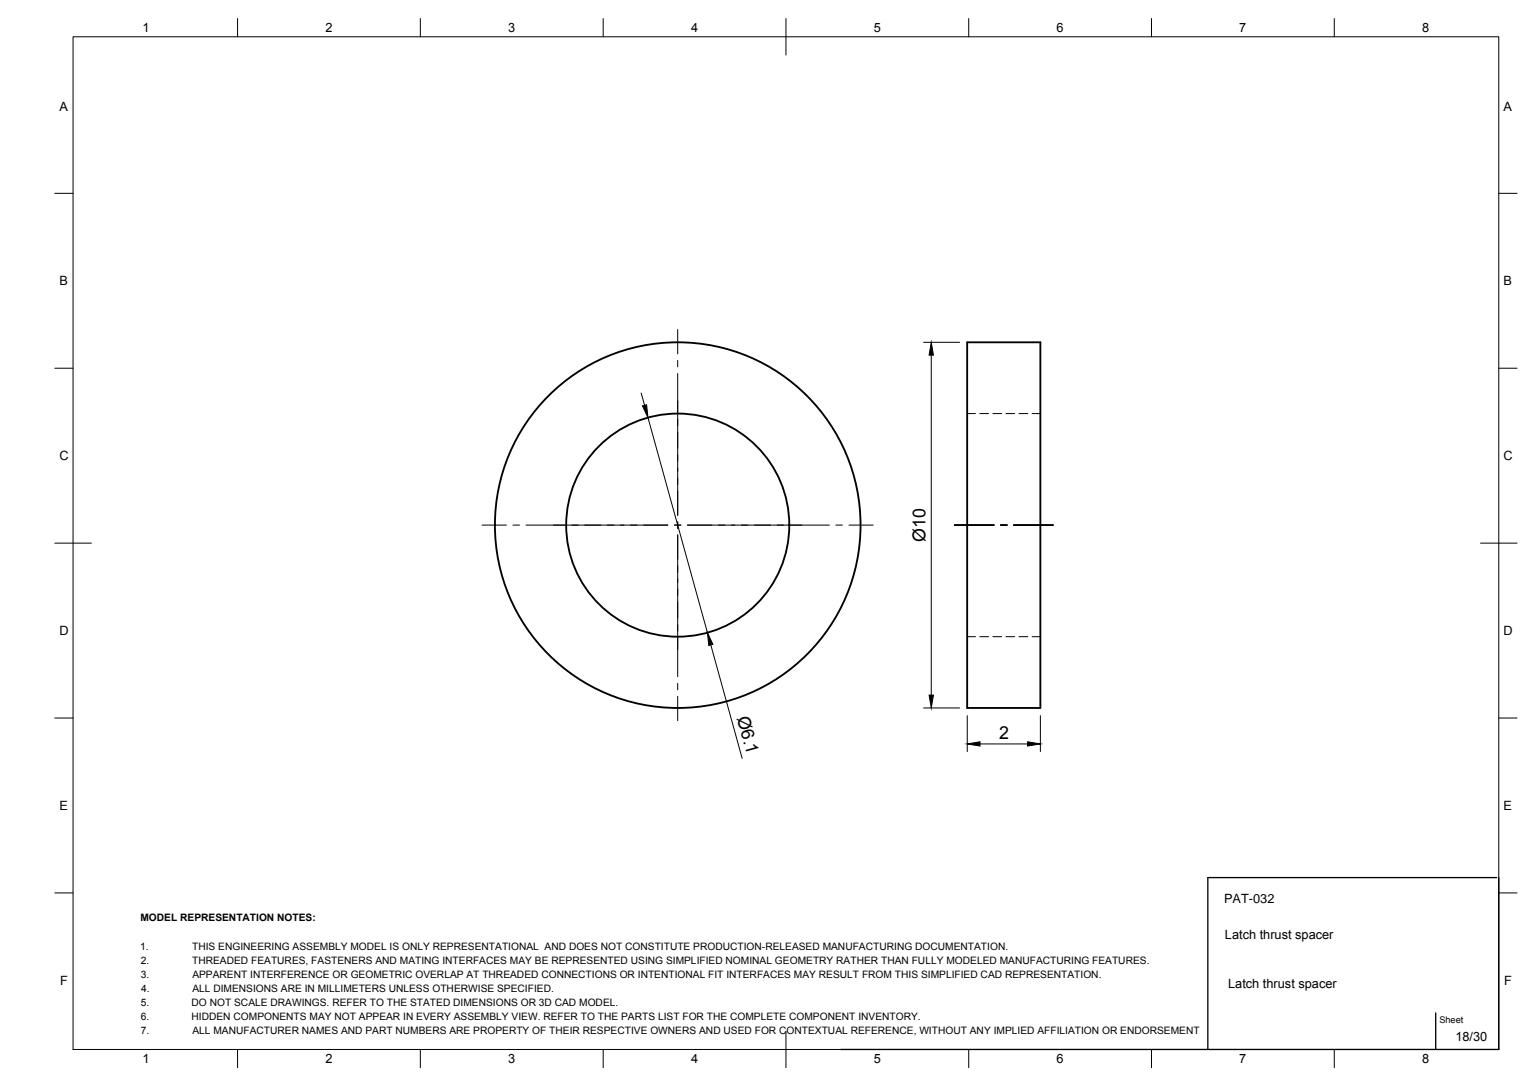
ISO-10303-21;
HEADER;
/* Generated by software containing ST-Developer
 * from STEP Tools, Inc. (www.steptools.com) 
 */

FILE_DESCRIPTION(
/* description */ ('Drill jig with bushing plate'),
/* implementation_level */ '2;1');

FILE_NAME(
/* name */ 'Latch thrust spacer.step',
/* time_stamp */ '2026-10-27T10:51:08-07:00',
/* author */ (''),
/* organization */ (''),
/* preprocessor_version */ 'ST-DEVELOPER v20.2',
/* originating_system */ 'Autodesk Translation Framework v15.17.0.0',
/* authorisation */ '');

FILE_SCHEMA (('AUTOMOTIVE_DESIGN { 1 0 10303 214 3 1 1 }'));
ENDSEC;

DATA;
#10=MECHANICAL_DESIGN_GEOMETRIC_PRESENTATION_REPRESENTATION('',(#236),#6638);
#188=SHAPE_REPRESENTATION_RELATIONSHIP('SRR','None',#6752,#212);
#212=ADVANCED_BREP_SHAPE_REPRESENTATION('',(#260),#6625);
#236=STYLED_ITEM('',(#6936),#260);
#260=MANIFOLD_SOLID_BREP('Body1',#3603);
#339=FACE_BOUND('',#903,.T.);
#340=FACE_BOUND('',#905,.T.);
#438=PLANE('',#4120);
#439=PLANE('',#4121);
#616=FACE_OUTER_BOUND('',#900,.T.);
#617=FACE_OUTER_BOUND('',#901,.T.);
#618=FACE_OUTER_BOUND('',#902,.T.);
#619=FACE_OUTER_BOUND('',#904,.T.);
#900=EDGE_LOOP('',(#2915,#2916,#2917,#2918));
#901=EDGE_LOOP('',(#2919,#2920,#2921,#2922));
#902=EDGE_LOOP('',(#2923));
#903=EDGE_LOOP('',(#2924));
#904=EDGE_LOOP('',(#2925));
#905=EDGE_LOOP('',(#2926));
#1165=LINE('',#6118,#1426);
#1166=LINE('',#6124,#1427);
#1426=VECTOR('',#4934,0.305);
#1427=VECTOR('',#4941,0.5);
#1654=CIRCLE('',#4115,0.305);
#1655=CIRCLE('',#4116,0.305);
#1656=CIRCLE('',#4118,0.5);
#1657=CIRCLE('',#4119,0.5);
#1880=VERTEX_POINT('',#6115);
#1881=VERTEX_POINT('',#6117);
#1882=VERTEX_POINT('',#6121);
#1883=VERTEX_POINT('',#6123);
#2245=EDGE_CURVE('',#1880,#1880,#1654,.T.);
#2246=EDGE_CURVE('',#1880,#1881,#1165,.T.);
#2247=EDGE_CURVE('',#1881,#1881,#1655,.T.);
#2248=EDGE_CURVE('',#1882,#1882,#1656,.T.);
#2249=EDGE_CURVE('',#1882,#1883,#1166,.T.);
#2250=EDGE_CURVE('',#1883,#1883,#1657,.T.);
#2915=ORIENTED_EDGE('',*,*,#2245,.F.);
#2916=ORIENTED_EDGE('',*,*,#2246,.T.);
#2917=ORIENTED_EDGE('',*,*,#2247,.T.);
#2918=ORIENTED_EDGE('',*,*,#2246,.F.);
#2919=ORIENTED_EDGE('',*,*,#2248,.F.);
#2920=ORIENTED_EDGE('',*,*,#2249,.T.);
#2921=ORIENTED_EDGE('',*,*,#2250,.T.);
#2922=ORIENTED_EDGE('',*,*,#2249,.F.);
#2923=ORIENTED_EDGE('',*,*,#2248,.T.);
#2924=ORIENTED_EDGE('',*,*,#2245,.T.);
#2925=ORIENTED_EDGE('',*,*,#2250,.F.);
#2926=ORIENTED_EDGE('',*,*,#2247,.F.);
#3346=CYLINDRICAL_SURFACE('',#4114,0.305);
#3347=CYLINDRICAL_SURFACE('',#4117,0.5);
#3491=ADVANCED_FACE('',(#616),#3346,.F.);
#3492=ADVANCED_FACE('',(#617),#3347,.T.);
#3493=ADVANCED_FACE('',(#618,#339),#438,.T.);
#3494=ADVANCED_FACE('',(#619,#340),#439,.F.);
#3603=CLOSED_SHELL('',(#3491,#3492,#3493,#3494));
#4113=AXIS2_PLACEMENT_3D('',#6113,#4928,#4929);
#4114=AXIS2_PLACEMENT_3D('',#6114,#4930,#4931);
#4115=AXIS2_PLACEMENT_3D('',#6116,#4932,#4933);
#4116=AXIS2_PLACEMENT_3D('',#6119,#4935,#4936);
#4117=AXIS2_PLACEMENT_3D('',#6120,#4937,#4938);
#4118=AXIS2_PLACEMENT_3D('',#6122,#4939,#4940);
#4119=AXIS2_PLACEMENT_3D('',#6125,#4942,#4943);
#4120=AXIS2_PLACEMENT_3D('',#6126,#4944,#4945);
#4121=AXIS2_PLACEMENT_3D('',#6127,#4946,#4947);
#4928=DIRECTION('axis',(0.,0.,1.));
#4929=DIRECTION('refdir',(1.,0.,0.));
#4930=DIRECTION('center_axis',(0.,0.,1.));
#4931=DIRECTION('ref_axis',(1.,0.,0.));
#4932=DIRECTION('center_axis',(0.,0.,-1.));
#4933=DIRECTION('ref_axis',(1.,0.,0.));
#4934=DIRECTION('',(0.,0.,-1.));
#4935=DIRECTION('center_axis',(0.,0.,-1.));
#4936=DIRECTION('ref_axis',(1.,0.,0.));
#4937=DIRECTION('center_axis',(0.,0.,1.));
#4938=DIRECTION('ref_axis',(1.,0.,0.));
#4939=DIRECTION('center_axis',(0.,0.,1.));
#4940=DIRECTION('ref_axis',(1.,0.,0.));
#4941=DIRECTION('',(0.,0.,-1.));
#4942=DIRECTION('center_axis',(0.,0.,1.));
#4943=DIRECTION('ref_axis',(1.,0.,0.));
#4944=DIRECTION('center_axis',(0.,0.,1.));
#4945=DIRECTION('ref_axis',(1.,0.,0.));
#4946=DIRECTION('center_axis',(0.,0.,1.));
#4947=DIRECTION('ref_axis',(1.,0.,0.));
#6113=CARTESIAN_POINT('',(0.,0.,0.));
#6114=CARTESIAN_POINT('Origin',(9.2,3.5,4.8));
#6115=CARTESIAN_POINT('',(8.895,3.5,5.));
#6116=CARTESIAN_POINT('Origin',(9.2,3.5,5.));
#6117=CARTESIAN_POINT('',(8.895,3.5,4.8));
#6118=CARTESIAN_POINT('',(8.895,3.5,4.8));
#6119=CARTESIAN_POINT('Origin',(9.2,3.5,4.8));
#6120=CARTESIAN_POINT('Origin',(9.2,3.5,4.8));
#6121=CARTESIAN_POINT('',(8.7,3.5,5.));
#6122=CARTESIAN_POINT('Origin',(9.2,3.5,5.));
#6123=CARTESIAN_POINT('',(8.7,3.5,4.8));
#6124=CARTESIAN_POINT('',(8.7,3.5,4.8));
#6125=CARTESIAN_POINT('Origin',(9.2,3.5,4.8));
#6126=CARTESIAN_POINT('Origin',(9.2,3.5,5.));
#6127=CARTESIAN_POINT('Origin',(9.2,3.5,4.8));
#6596=UNCERTAINTY_MEASURE_WITH_UNIT(LENGTH_MEASURE(0.001),#6639,
'DISTANCE_ACCURACY_VALUE',
'Maximum model space distance between geometric entities at asserted c
onnectivities');
#6609=UNCERTAINTY_MEASURE_WITH_UNIT(LENGTH_MEASURE(0.001),#6639,
'DISTANCE_ACCURACY_VALUE',
'Maximum model space distance between geometric entities at asserted c
onnectivities');
#6625=(
GEOMETRIC_REPRESENTATION_CONTEXT(3)
GLOBAL_UNCERTAINTY_ASSIGNED_CONTEXT((#6596))
GLOBAL_UNIT_ASSIGNED_CONTEXT((#6639,#6641,#6642))
REPRESENTATION_CONTEXT('','3D')
);
#6638=(
GEOMETRIC_REPRESENTATION_CONTEXT(3)
GLOBAL_UNCERTAINTY_ASSIGNED_CONTEXT((#6609))
GLOBAL_UNIT_ASSIGNED_CONTEXT((#6639,#6641,#6642))
REPRESENTATION_CONTEXT('','3D')
);
#6639=(
LENGTH_UNIT()
NAMED_UNIT(*)
SI_UNIT(.CENTI.,.METRE.)
);
#6641=(
NAMED_UNIT(*)
PLANE_ANGLE_UNIT()
SI_UNIT($,.RADIAN.)
);
#6642=(
NAMED_UNIT(*)
SI_UNIT($,.STERADIAN.)
SOLID_ANGLE_UNIT()
);
#6658=SHAPE_DEFINITION_REPRESENTATION(#6686,#6752);
#6686=PRODUCT_DEFINITION_SHAPE('',$,#6781);
#6752=SHAPE_REPRESENTATION('',(#4113),#6625);
#6765=PRODUCT_DEFINITION_CONTEXT('part definition',#6851,'design');
#6781=PRODUCT_DEFINITION('Latch thrust spacer','Latch thrust spacer',#6809,
#6765);
#6809=PRODUCT_DEFINITION_FORMATION('',$,#6868);
#6851=APPLICATION_CONTEXT(
'Core Data for Automotive Mechanical Design Process');
#6852=PRODUCT_CONTEXT('part definition',#6851,'mechanical');
#6868=PRODUCT('Latch thrust spacer','Latch thrust spacer',
'Latch thrust spacer',(#6852));
#6930=COLOUR_RGB('Sky Blue',0.24,0.69,0.87);
#6931=FILL_AREA_STYLE_COLOUR('',#6930);
#6932=FILL_AREA_STYLE('',(#6931));
#6933=SURFACE_STYLE_FILL_AREA(#6932);
#6934=SURFACE_SIDE_STYLE('',(#6933));
#6935=SURFACE_STYLE_USAGE(.BOTH.,#6934);
#6936=PRESENTATION_STYLE_ASSIGNMENT((#6935));
ENDSEC;
END-ISO-10303-21;
